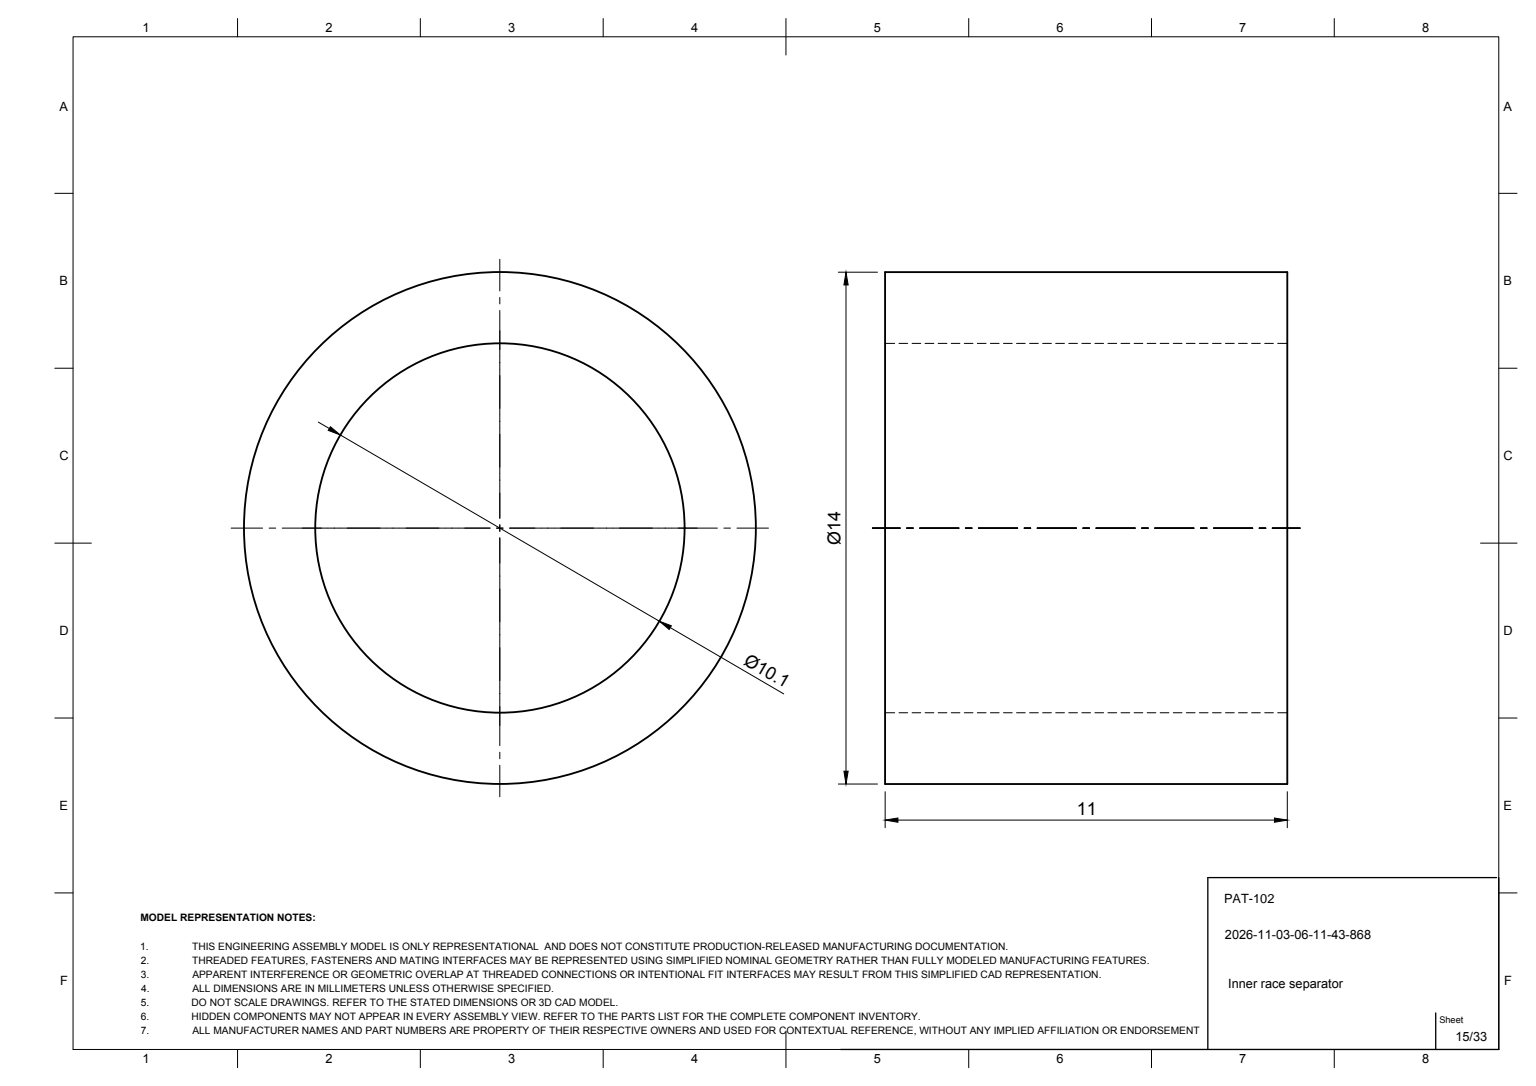
ISO-10303-21;
HEADER;
/* Generated by software containing ST-Developer
 * from STEP Tools, Inc. (www.steptools.com) 
 */

FILE_DESCRIPTION(
/* description */ ('Swing-away clamp arm'),
/* implementation_level */ '2;1');

FILE_NAME(
/* name */ 'Inner race separator.step',
/* time_stamp */ '2026-10-28T03:26:03-07:00',
/* author */ (''),
/* organization */ (''),
/* preprocessor_version */ 'ST-DEVELOPER v20.2',
/* originating_system */ 'Autodesk Translation Framework v15.17.0.0',
/* authorisation */ '');

FILE_SCHEMA (('AUTOMOTIVE_DESIGN { 1 0 10303 214 3 1 1 }'));
ENDSEC;

DATA;
#10=MECHANICAL_DESIGN_GEOMETRIC_PRESENTATION_REPRESENTATION('',(#302),#10627);
#250=SHAPE_REPRESENTATION_RELATIONSHIP('SRR','None',#10749,#276);
#276=ADVANCED_BREP_SHAPE_REPRESENTATION('',(#335),#10608);
#302=STYLED_ITEM('',(#10965),#335);
#335=MANIFOLD_SOLID_BREP('Body1',#4909);
#399=FACE_BOUND('',#1123,.T.);
#400=FACE_BOUND('',#1125,.T.);
#554=PLANE('',#5476);
#555=PLANE('',#5477);
#772=FACE_OUTER_BOUND('',#1120,.T.);
#773=FACE_OUTER_BOUND('',#1121,.T.);
#774=FACE_OUTER_BOUND('',#1122,.T.);
#775=FACE_OUTER_BOUND('',#1124,.T.);
#1120=EDGE_LOOP('',(#3861,#3862,#3863,#3864));
#1121=EDGE_LOOP('',(#3865,#3866,#3867,#3868));
#1122=EDGE_LOOP('',(#3869));
#1123=EDGE_LOOP('',(#3870));
#1124=EDGE_LOOP('',(#3871));
#1125=EDGE_LOOP('',(#3872));
#1550=LINE('',#9470,#1872);
#1551=LINE('',#9476,#1873);
#1872=VECTOR('',#6567,0.505);
#1873=VECTOR('',#6574,0.7);
#2085=CIRCLE('',#5471,0.505);
#2086=CIRCLE('',#5472,0.505);
#2087=CIRCLE('',#5474,0.7);
#2088=CIRCLE('',#5475,0.7);
#2454=VERTEX_POINT('',#9467);
#2455=VERTEX_POINT('',#9469);
#2456=VERTEX_POINT('',#9473);
#2457=VERTEX_POINT('',#9475);
#2963=EDGE_CURVE('',#2454,#2454,#2085,.T.);
#2964=EDGE_CURVE('',#2454,#2455,#1550,.T.);
#2965=EDGE_CURVE('',#2455,#2455,#2086,.T.);
#2966=EDGE_CURVE('',#2456,#2456,#2087,.T.);
#2967=EDGE_CURVE('',#2456,#2457,#1551,.T.);
#2968=EDGE_CURVE('',#2457,#2457,#2088,.T.);
#3861=ORIENTED_EDGE('',*,*,#2963,.F.);
#3862=ORIENTED_EDGE('',*,*,#2964,.T.);
#3863=ORIENTED_EDGE('',*,*,#2965,.T.);
#3864=ORIENTED_EDGE('',*,*,#2964,.F.);
#3865=ORIENTED_EDGE('',*,*,#2966,.F.);
#3866=ORIENTED_EDGE('',*,*,#2967,.T.);
#3867=ORIENTED_EDGE('',*,*,#2968,.T.);
#3868=ORIENTED_EDGE('',*,*,#2967,.F.);
#3869=ORIENTED_EDGE('',*,*,#2966,.T.);
#3870=ORIENTED_EDGE('',*,*,#2963,.T.);
#3871=ORIENTED_EDGE('',*,*,#2968,.F.);
#3872=ORIENTED_EDGE('',*,*,#2965,.F.);
#4532=CYLINDRICAL_SURFACE('',#5470,0.505);
#4533=CYLINDRICAL_SURFACE('',#5473,0.7);
#4727=ADVANCED_FACE('',(#772),#4532,.F.);
#4728=ADVANCED_FACE('',(#773),#4533,.T.);
#4729=ADVANCED_FACE('',(#774,#399),#554,.T.);
#4730=ADVANCED_FACE('',(#775,#400),#555,.F.);
#4909=CLOSED_SHELL('',(#4727,#4728,#4729,#4730));
#5469=AXIS2_PLACEMENT_3D('',#9465,#6561,#6562);
#5470=AXIS2_PLACEMENT_3D('',#9466,#6563,#6564);
#5471=AXIS2_PLACEMENT_3D('',#9468,#6565,#6566);
#5472=AXIS2_PLACEMENT_3D('',#9471,#6568,#6569);
#5473=AXIS2_PLACEMENT_3D('',#9472,#6570,#6571);
#5474=AXIS2_PLACEMENT_3D('',#9474,#6572,#6573);
#5475=AXIS2_PLACEMENT_3D('',#9477,#6575,#6576);
#5476=AXIS2_PLACEMENT_3D('',#9478,#6577,#6578);
#5477=AXIS2_PLACEMENT_3D('',#9479,#6579,#6580);
#6561=DIRECTION('axis',(0.,0.,1.));
#6562=DIRECTION('refdir',(1.,0.,0.));
#6563=DIRECTION('center_axis',(0.,0.,1.));
#6564=DIRECTION('ref_axis',(1.,0.,0.));
#6565=DIRECTION('center_axis',(0.,0.,-1.));
#6566=DIRECTION('ref_axis',(1.,0.,0.));
#6567=DIRECTION('',(0.,0.,-1.));
#6568=DIRECTION('center_axis',(0.,0.,-1.));
#6569=DIRECTION('ref_axis',(1.,0.,0.));
#6570=DIRECTION('center_axis',(0.,0.,1.));
#6571=DIRECTION('ref_axis',(1.,0.,0.));
#6572=DIRECTION('center_axis',(0.,0.,1.));
#6573=DIRECTION('ref_axis',(1.,0.,0.));
#6574=DIRECTION('',(0.,0.,-1.));
#6575=DIRECTION('center_axis',(0.,0.,1.));
#6576=DIRECTION('ref_axis',(1.,0.,0.));
#6577=DIRECTION('center_axis',(0.,0.,1.));
#6578=DIRECTION('ref_axis',(1.,0.,0.));
#6579=DIRECTION('center_axis',(0.,0.,1.));
#6580=DIRECTION('ref_axis',(1.,0.,0.));
#9465=CARTESIAN_POINT('',(0.,0.,0.));
#9466=CARTESIAN_POINT('Origin',(0.,0.,6.95));
#9467=CARTESIAN_POINT('',(-0.505,-6.18446633569413E-17,8.05));
#9468=CARTESIAN_POINT('Origin',(0.,0.,8.05));
#9469=CARTESIAN_POINT('',(-0.505,-6.18446633569413E-17,6.95));
#9470=CARTESIAN_POINT('',(-0.505,-6.18446633569413E-17,6.95));
#9471=CARTESIAN_POINT('Origin',(0.,0.,6.95));
#9472=CARTESIAN_POINT('Origin',(0.,0.,6.95));
#9473=CARTESIAN_POINT('',(-0.7,-8.57252759403147E-17,8.05));
#9474=CARTESIAN_POINT('Origin',(0.,0.,8.05));
#9475=CARTESIAN_POINT('',(-0.7,-8.57252759403147E-17,6.95));
#9476=CARTESIAN_POINT('',(-0.7,-8.57252759403147E-17,6.95));
#9477=CARTESIAN_POINT('Origin',(0.,0.,6.95));
#9478=CARTESIAN_POINT('Origin',(0.,0.,8.05));
#9479=CARTESIAN_POINT('Origin',(0.,0.,6.95));
#10576=UNCERTAINTY_MEASURE_WITH_UNIT(LENGTH_MEASURE(0.001),#10628,
'DISTANCE_ACCURACY_VALUE',
'Maximum model space distance between geometric entities at asserted c
onnectivities');
#10595=UNCERTAINTY_MEASURE_WITH_UNIT(LENGTH_MEASURE(0.001),#10628,
'DISTANCE_ACCURACY_VALUE',
'Maximum model space distance between geometric entities at asserted c
onnectivities');
#10608=(
GEOMETRIC_REPRESENTATION_CONTEXT(3)
GLOBAL_UNCERTAINTY_ASSIGNED_CONTEXT((#10576))
GLOBAL_UNIT_ASSIGNED_CONTEXT((#10628,#10630,#10631))
REPRESENTATION_CONTEXT('','3D')
);
#10627=(
GEOMETRIC_REPRESENTATION_CONTEXT(3)
GLOBAL_UNCERTAINTY_ASSIGNED_CONTEXT((#10595))
GLOBAL_UNIT_ASSIGNED_CONTEXT((#10628,#10630,#10631))
REPRESENTATION_CONTEXT('','3D')
);
#10628=(
LENGTH_UNIT()
NAMED_UNIT(*)
SI_UNIT(.CENTI.,.METRE.)
);
#10630=(
NAMED_UNIT(*)
PLANE_ANGLE_UNIT()
SI_UNIT($,.RADIAN.)
);
#10631=(
NAMED_UNIT(*)
SI_UNIT($,.STERADIAN.)
SOLID_ANGLE_UNIT()
);
#10644=SHAPE_DEFINITION_REPRESENTATION(#10685,#10749);
#10685=PRODUCT_DEFINITION_SHAPE('',$,#10781);
#10749=SHAPE_REPRESENTATION('',(#5469),#10608);
#10768=PRODUCT_DEFINITION_CONTEXT('part definition',#10863,'design');
#10781=PRODUCT_DEFINITION('Inner race separator','Inner race separator',
#10812,#10768);
#10812=PRODUCT_DEFINITION_FORMATION('',$,#10877);
#10863=APPLICATION_CONTEXT(
'Core Data for Automotive Mechanical Design Process');
#10864=PRODUCT_CONTEXT('part definition',#10863,'mechanical');
#10877=PRODUCT('Inner race separator','Inner race separator',
'Inner race separator',(#10864));
#10959=COLOUR_RGB('Grey',0.48,0.52,0.57);
#10960=FILL_AREA_STYLE_COLOUR('',#10959);
#10961=FILL_AREA_STYLE('',(#10960));
#10962=SURFACE_STYLE_FILL_AREA(#10961);
#10963=SURFACE_SIDE_STYLE('',(#10962));
#10964=SURFACE_STYLE_USAGE(.BOTH.,#10963);
#10965=PRESENTATION_STYLE_ASSIGNMENT((#10964));
ENDSEC;
END-ISO-10303-21;
